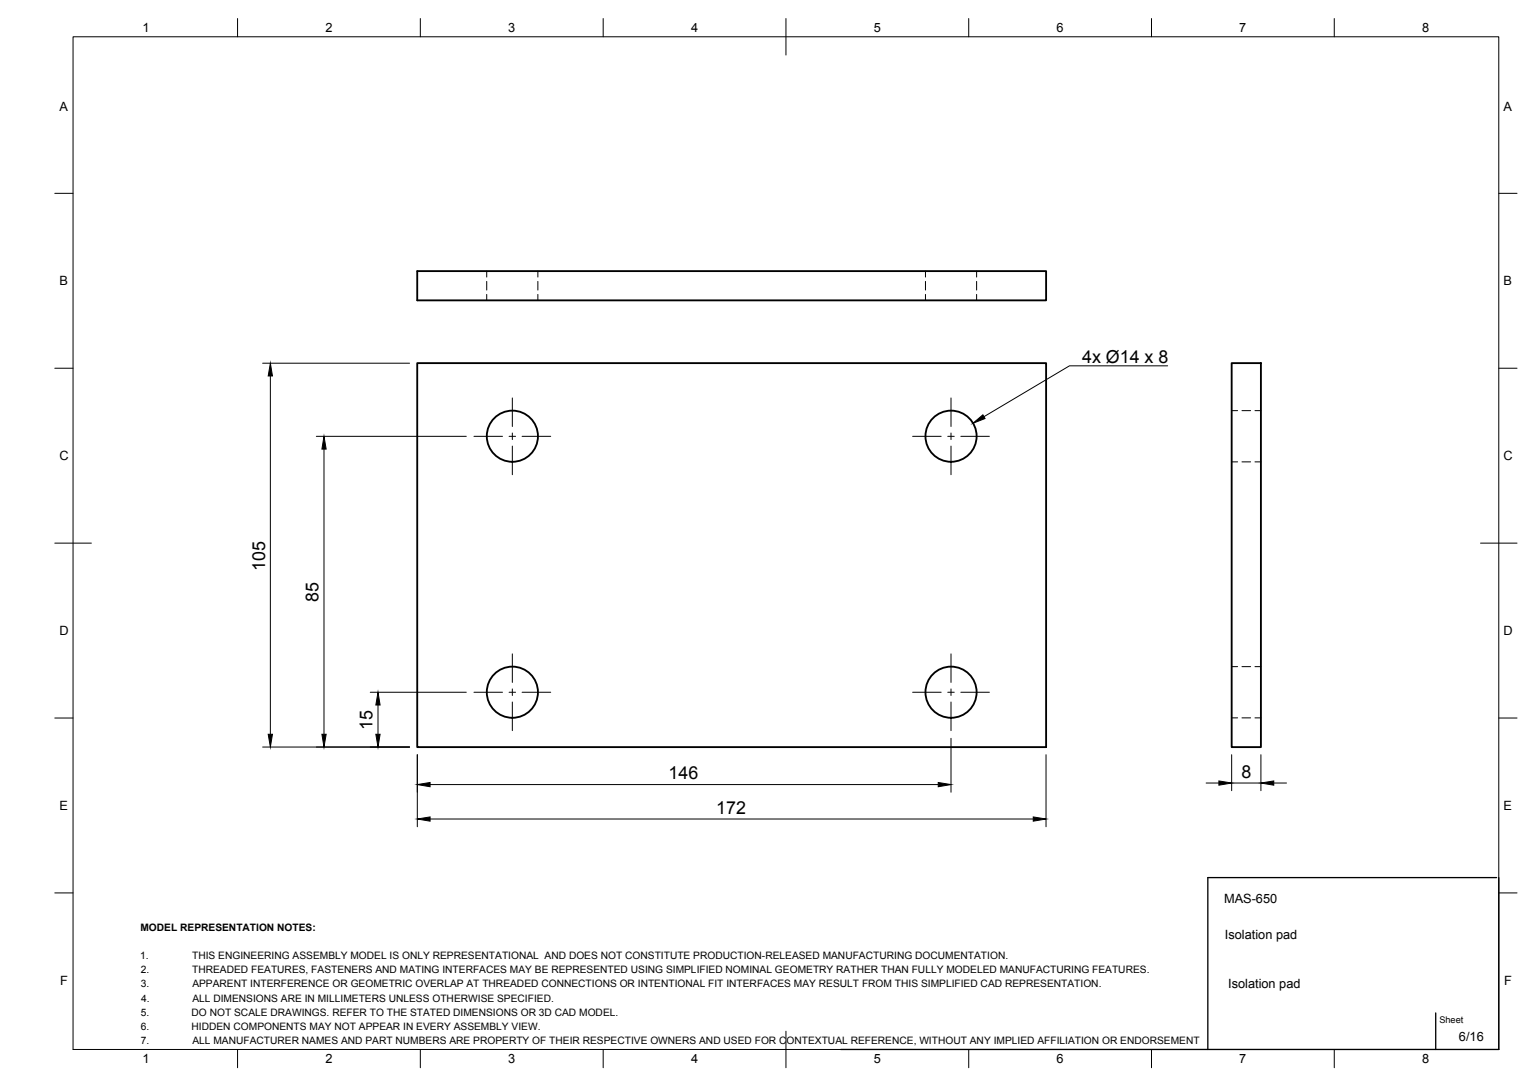
ISO-10303-21;
HEADER;
/* Generated by software containing ST-Developer
 * from STEP Tools, Inc. (www.steptools.com) 
 */

FILE_DESCRIPTION(
/* description */ ('Independent manual traversing gantry with native reusable aluminum pr
ofiles,180mm captured carriage travel, four bronze-bushed rollers, lin
ked ideal rolling motion, bonded acetal lateral guides, positive welde
d end stops and fully retained axle stacks. Editable native profile cu
t lengths220/400mm. Tool attachments viaM6 bridge-plate taps; mounted 
tool outside assembly. Welds, anchors, adhesives, fits, traction, load
/speed/structural/life ratings unassigned.'),
/* implementation_level */ '2;1');

FILE_NAME(
/* name */ 'Isolation pad.step',
/* time_stamp */ '2026-11-09T20:04:38-08:00',
/* author */ (''),
/* organization */ (''),
/* preprocessor_version */ 'ST-DEVELOPER v20.2',
/* originating_system */ 'Autodesk Translation Framework v15.17.0.0',
/* authorisation */ '');

FILE_SCHEMA (('AUTOMOTIVE_DESIGN { 1 0 10303 214 3 1 1 }'));
ENDSEC;

DATA;
#10=MECHANICAL_DESIGN_GEOMETRIC_PRESENTATION_REPRESENTATION('',(#474),#13231);
#442=SHAPE_REPRESENTATION_RELATIONSHIP('SRR','None',#13331,#458);
#458=ADVANCED_BREP_SHAPE_REPRESENTATION('',(#490),#13218);
#474=STYLED_ITEM('',(#13420),#490);
#490=MANIFOLD_SOLID_BREP('Body1',#4154);
#515=FACE_BOUND('',#921,.T.);
#516=FACE_BOUND('',#922,.T.);
#517=FACE_BOUND('',#923,.T.);
#518=FACE_BOUND('',#924,.T.);
#519=FACE_BOUND('',#926,.T.);
#520=FACE_BOUND('',#927,.T.);
#521=FACE_BOUND('',#928,.T.);
#522=FACE_BOUND('',#929,.T.);
#578=PLANE('',#4447);
#579=PLANE('',#4448);
#580=PLANE('',#4449);
#581=PLANE('',#4450);
#582=PLANE('',#4451);
#583=PLANE('',#4452);
#679=FACE_OUTER_BOUND('',#912,.T.);
#680=FACE_OUTER_BOUND('',#913,.T.);
#681=FACE_OUTER_BOUND('',#914,.T.);
#682=FACE_OUTER_BOUND('',#915,.T.);
#683=FACE_OUTER_BOUND('',#916,.T.);
#684=FACE_OUTER_BOUND('',#917,.T.);
#685=FACE_OUTER_BOUND('',#918,.T.);
#686=FACE_OUTER_BOUND('',#919,.T.);
#687=FACE_OUTER_BOUND('',#920,.T.);
#688=FACE_OUTER_BOUND('',#925,.T.);
#912=EDGE_LOOP('',(#2922,#2923,#2924,#2925));
#913=EDGE_LOOP('',(#2926,#2927,#2928,#2929));
#914=EDGE_LOOP('',(#2930,#2931,#2932,#2933));
#915=EDGE_LOOP('',(#2934,#2935,#2936,#2937));
#916=EDGE_LOOP('',(#2938,#2939,#2940,#2941));
#917=EDGE_LOOP('',(#2942,#2943,#2944,#2945));
#918=EDGE_LOOP('',(#2946,#2947,#2948,#2949));
#919=EDGE_LOOP('',(#2950,#2951,#2952,#2953));
#920=EDGE_LOOP('',(#2954,#2955,#2956,#2957));
#921=EDGE_LOOP('',(#2958));
#922=EDGE_LOOP('',(#2959));
#923=EDGE_LOOP('',(#2960));
#924=EDGE_LOOP('',(#2961));
#925=EDGE_LOOP('',(#2962,#2963,#2964,#2965));
#926=EDGE_LOOP('',(#2966));
#927=EDGE_LOOP('',(#2967));
#928=EDGE_LOOP('',(#2968));
#929=EDGE_LOOP('',(#2969));
#1204=LINE('',#6034,#1466);
#1205=LINE('',#6040,#1467);
#1206=LINE('',#6046,#1468);
#1207=LINE('',#6052,#1469);
#1208=LINE('',#6057,#1470);
#1209=LINE('',#6059,#1471);
#1210=LINE('',#6061,#1472);
#1211=LINE('',#6062,#1473);
#1212=LINE('',#6065,#1474);
#1213=LINE('',#6067,#1475);
#1214=LINE('',#6068,#1476);
#1215=LINE('',#6071,#1477);
#1216=LINE('',#6073,#1478);
#1217=LINE('',#6074,#1479);
#1218=LINE('',#6076,#1480);
#1219=LINE('',#6077,#1481);
#1466=VECTOR('',#5001,7.);
#1467=VECTOR('',#5008,7.);
#1468=VECTOR('',#5015,7.);
#1469=VECTOR('',#5022,7.);
#1470=VECTOR('',#5027,10.);
#1471=VECTOR('',#5028,10.);
#1472=VECTOR('',#5029,10.);
#1473=VECTOR('',#5030,10.);
#1474=VECTOR('',#5033,10.);
#1475=VECTOR('',#5034,10.);
#1476=VECTOR('',#5035,10.);
#1477=VECTOR('',#5038,10.);
#1478=VECTOR('',#5039,10.);
#1479=VECTOR('',#5040,10.);
#1480=VECTOR('',#5043,10.);
#1481=VECTOR('',#5044,10.);
#1688=CIRCLE('',#4436,7.);
#1689=CIRCLE('',#4437,7.);
#1690=CIRCLE('',#4439,7.);
#1691=CIRCLE('',#4440,7.);
#1692=CIRCLE('',#4442,7.);
#1693=CIRCLE('',#4443,7.);
#1694=CIRCLE('',#4445,7.);
#1695=CIRCLE('',#4446,7.);
#1832=VERTEX_POINT('',#6031);
#1833=VERTEX_POINT('',#6033);
#1834=VERTEX_POINT('',#6037);
#1835=VERTEX_POINT('',#6039);
#1836=VERTEX_POINT('',#6043);
#1837=VERTEX_POINT('',#6045);
#1838=VERTEX_POINT('',#6049);
#1839=VERTEX_POINT('',#6051);
#1840=VERTEX_POINT('',#6055);
#1841=VERTEX_POINT('',#6056);
#1842=VERTEX_POINT('',#6058);
#1843=VERTEX_POINT('',#6060);
#1844=VERTEX_POINT('',#6064);
#1845=VERTEX_POINT('',#6066);
#1846=VERTEX_POINT('',#6070);
#1847=VERTEX_POINT('',#6072);
#2244=EDGE_CURVE('',#1832,#1832,#1688,.T.);
#2245=EDGE_CURVE('',#1832,#1833,#1204,.T.);
#2246=EDGE_CURVE('',#1833,#1833,#1689,.T.);
#2247=EDGE_CURVE('',#1834,#1834,#1690,.T.);
#2248=EDGE_CURVE('',#1834,#1835,#1205,.T.);
#2249=EDGE_CURVE('',#1835,#1835,#1691,.T.);
#2250=EDGE_CURVE('',#1836,#1836,#1692,.T.);
#2251=EDGE_CURVE('',#1836,#1837,#1206,.T.);
#2252=EDGE_CURVE('',#1837,#1837,#1693,.T.);
#2253=EDGE_CURVE('',#1838,#1838,#1694,.T.);
#2254=EDGE_CURVE('',#1838,#1839,#1207,.T.);
#2255=EDGE_CURVE('',#1839,#1839,#1695,.T.);
#2256=EDGE_CURVE('',#1840,#1841,#1208,.F.);
#2257=EDGE_CURVE('',#1841,#1842,#1209,.T.);
#2258=EDGE_CURVE('',#1843,#1842,#1210,.F.);
#2259=EDGE_CURVE('',#1840,#1843,#1211,.T.);
#2260=EDGE_CURVE('',#1844,#1840,#1212,.F.);
#2261=EDGE_CURVE('',#1845,#1843,#1213,.F.);
#2262=EDGE_CURVE('',#1844,#1845,#1214,.T.);
#2263=EDGE_CURVE('',#1846,#1844,#1215,.F.);
#2264=EDGE_CURVE('',#1847,#1845,#1216,.F.);
#2265=EDGE_CURVE('',#1846,#1847,#1217,.F.);
#2266=EDGE_CURVE('',#1841,#1846,#1218,.T.);
#2267=EDGE_CURVE('',#1842,#1847,#1219,.T.);
#2922=ORIENTED_EDGE('',*,*,#2244,.F.);
#2923=ORIENTED_EDGE('',*,*,#2245,.T.);
#2924=ORIENTED_EDGE('',*,*,#2246,.F.);
#2925=ORIENTED_EDGE('',*,*,#2245,.F.);
#2926=ORIENTED_EDGE('',*,*,#2247,.F.);
#2927=ORIENTED_EDGE('',*,*,#2248,.T.);
#2928=ORIENTED_EDGE('',*,*,#2249,.F.);
#2929=ORIENTED_EDGE('',*,*,#2248,.F.);
#2930=ORIENTED_EDGE('',*,*,#2250,.F.);
#2931=ORIENTED_EDGE('',*,*,#2251,.T.);
#2932=ORIENTED_EDGE('',*,*,#2252,.F.);
#2933=ORIENTED_EDGE('',*,*,#2251,.F.);
#2934=ORIENTED_EDGE('',*,*,#2253,.F.);
#2935=ORIENTED_EDGE('',*,*,#2254,.T.);
#2936=ORIENTED_EDGE('',*,*,#2255,.F.);
#2937=ORIENTED_EDGE('',*,*,#2254,.F.);
#2938=ORIENTED_EDGE('',*,*,#2256,.T.);
#2939=ORIENTED_EDGE('',*,*,#2257,.T.);
#2940=ORIENTED_EDGE('',*,*,#2258,.F.);
#2941=ORIENTED_EDGE('',*,*,#2259,.F.);
#2942=ORIENTED_EDGE('',*,*,#2260,.T.);
#2943=ORIENTED_EDGE('',*,*,#2259,.T.);
#2944=ORIENTED_EDGE('',*,*,#2261,.F.);
#2945=ORIENTED_EDGE('',*,*,#2262,.F.);
#2946=ORIENTED_EDGE('',*,*,#2263,.T.);
#2947=ORIENTED_EDGE('',*,*,#2262,.T.);
#2948=ORIENTED_EDGE('',*,*,#2264,.F.);
#2949=ORIENTED_EDGE('',*,*,#2265,.F.);
#2950=ORIENTED_EDGE('',*,*,#2266,.T.);
#2951=ORIENTED_EDGE('',*,*,#2265,.T.);
#2952=ORIENTED_EDGE('',*,*,#2267,.F.);
#2953=ORIENTED_EDGE('',*,*,#2257,.F.);
#2954=ORIENTED_EDGE('',*,*,#2267,.T.);
#2955=ORIENTED_EDGE('',*,*,#2264,.T.);
#2956=ORIENTED_EDGE('',*,*,#2261,.T.);
#2957=ORIENTED_EDGE('',*,*,#2258,.T.);
#2958=ORIENTED_EDGE('',*,*,#2244,.T.);
#2959=ORIENTED_EDGE('',*,*,#2247,.T.);
#2960=ORIENTED_EDGE('',*,*,#2250,.T.);
#2961=ORIENTED_EDGE('',*,*,#2253,.T.);
#2962=ORIENTED_EDGE('',*,*,#2266,.F.);
#2963=ORIENTED_EDGE('',*,*,#2256,.F.);
#2964=ORIENTED_EDGE('',*,*,#2260,.F.);
#2965=ORIENTED_EDGE('',*,*,#2263,.F.);
#2966=ORIENTED_EDGE('',*,*,#2246,.T.);
#2967=ORIENTED_EDGE('',*,*,#2249,.T.);
#2968=ORIENTED_EDGE('',*,*,#2252,.T.);
#2969=ORIENTED_EDGE('',*,*,#2255,.T.);
#3818=CYLINDRICAL_SURFACE('',#4435,7.);
#3819=CYLINDRICAL_SURFACE('',#4438,7.);
#3820=CYLINDRICAL_SURFACE('',#4441,7.);
#3821=CYLINDRICAL_SURFACE('',#4444,7.);
#3976=ADVANCED_FACE('',(#679),#3818,.F.);
#3977=ADVANCED_FACE('',(#680),#3819,.F.);
#3978=ADVANCED_FACE('',(#681),#3820,.F.);
#3979=ADVANCED_FACE('',(#682),#3821,.F.);
#3980=ADVANCED_FACE('',(#683),#578,.T.);
#3981=ADVANCED_FACE('',(#684),#579,.T.);
#3982=ADVANCED_FACE('',(#685),#580,.T.);
#3983=ADVANCED_FACE('',(#686),#581,.T.);
#3984=ADVANCED_FACE('',(#687,#515,#516,#517,#518),#582,.T.);
#3985=ADVANCED_FACE('',(#688,#519,#520,#521,#522),#583,.F.);
#4154=CLOSED_SHELL('',(#3976,#3977,#3978,#3979,#3980,#3981,#3982,#3983,
#3984,#3985));
#4434=AXIS2_PLACEMENT_3D('',#6029,#4995,#4996);
#4435=AXIS2_PLACEMENT_3D('',#6030,#4997,#4998);
#4436=AXIS2_PLACEMENT_3D('',#6032,#4999,#5000);
#4437=AXIS2_PLACEMENT_3D('',#6035,#5002,#5003);
#4438=AXIS2_PLACEMENT_3D('',#6036,#5004,#5005);
#4439=AXIS2_PLACEMENT_3D('',#6038,#5006,#5007);
#4440=AXIS2_PLACEMENT_3D('',#6041,#5009,#5010);
#4441=AXIS2_PLACEMENT_3D('',#6042,#5011,#5012);
#4442=AXIS2_PLACEMENT_3D('',#6044,#5013,#5014);
#4443=AXIS2_PLACEMENT_3D('',#6047,#5016,#5017);
#4444=AXIS2_PLACEMENT_3D('',#6048,#5018,#5019);
#4445=AXIS2_PLACEMENT_3D('',#6050,#5020,#5021);
#4446=AXIS2_PLACEMENT_3D('',#6053,#5023,#5024);
#4447=AXIS2_PLACEMENT_3D('',#6054,#5025,#5026);
#4448=AXIS2_PLACEMENT_3D('',#6063,#5031,#5032);
#4449=AXIS2_PLACEMENT_3D('',#6069,#5036,#5037);
#4450=AXIS2_PLACEMENT_3D('',#6075,#5041,#5042);
#4451=AXIS2_PLACEMENT_3D('',#6078,#5045,#5046);
#4452=AXIS2_PLACEMENT_3D('',#6079,#5047,#5048);
#4995=DIRECTION('axis',(0.,0.,1.));
#4996=DIRECTION('refdir',(1.,0.,0.));
#4997=DIRECTION('center_axis',(0.,0.,-1.));
#4998=DIRECTION('ref_axis',(1.,0.,0.));
#4999=DIRECTION('center_axis',(0.,0.,-1.));
#5000=DIRECTION('ref_axis',(1.,0.,0.));
#5001=DIRECTION('',(0.,0.,-1.));
#5002=DIRECTION('center_axis',(0.,0.,1.));
#5003=DIRECTION('ref_axis',(1.,0.,0.));
#5004=DIRECTION('center_axis',(0.,0.,-1.));
#5005=DIRECTION('ref_axis',(1.,0.,0.));
#5006=DIRECTION('center_axis',(0.,0.,-1.));
#5007=DIRECTION('ref_axis',(1.,0.,0.));
#5008=DIRECTION('',(0.,0.,-1.));
#5009=DIRECTION('center_axis',(0.,0.,1.));
#5010=DIRECTION('ref_axis',(1.,0.,0.));
#5011=DIRECTION('center_axis',(0.,0.,-1.));
#5012=DIRECTION('ref_axis',(1.,0.,0.));
#5013=DIRECTION('center_axis',(0.,0.,-1.));
#5014=DIRECTION('ref_axis',(1.,0.,0.));
#5015=DIRECTION('',(0.,0.,-1.));
#5016=DIRECTION('center_axis',(0.,0.,1.));
#5017=DIRECTION('ref_axis',(1.,0.,0.));
#5018=DIRECTION('center_axis',(0.,0.,-1.));
#5019=DIRECTION('ref_axis',(1.,0.,0.));
#5020=DIRECTION('center_axis',(0.,0.,-1.));
#5021=DIRECTION('ref_axis',(1.,0.,0.));
#5022=DIRECTION('',(0.,0.,-1.));
#5023=DIRECTION('center_axis',(0.,0.,1.));
#5024=DIRECTION('ref_axis',(1.,0.,0.));
#5025=DIRECTION('center_axis',(0.,1.,0.));
#5026=DIRECTION('ref_axis',(-1.,0.,0.));
#5027=DIRECTION('',(1.,0.,0.));
#5028=DIRECTION('',(0.,0.,1.));
#5029=DIRECTION('',(1.,0.,0.));
#5030=DIRECTION('',(0.,0.,1.));
#5031=DIRECTION('center_axis',(1.,0.,0.));
#5032=DIRECTION('ref_axis',(0.,1.,0.));
#5033=DIRECTION('',(0.,-1.,0.));
#5034=DIRECTION('',(0.,-1.,0.));
#5035=DIRECTION('',(0.,0.,1.));
#5036=DIRECTION('center_axis',(0.,-1.,0.));
#5037=DIRECTION('ref_axis',(1.,0.,0.));
#5038=DIRECTION('',(-1.,0.,0.));
#5039=DIRECTION('',(-1.,0.,0.));
#5040=DIRECTION('',(0.,0.,-1.));
#5041=DIRECTION('center_axis',(-1.,0.,0.));
#5042=DIRECTION('ref_axis',(0.,-1.,0.));
#5043=DIRECTION('',(0.,-1.,0.));
#5044=DIRECTION('',(0.,-1.,0.));
#5045=DIRECTION('center_axis',(0.,0.,1.));
#5046=DIRECTION('ref_axis',(1.,0.,0.));
#5047=DIRECTION('center_axis',(0.,0.,1.));
#5048=DIRECTION('ref_axis',(1.,0.,0.));
#6029=CARTESIAN_POINT('',(0.,0.,0.));
#6030=CARTESIAN_POINT('Origin',(35.,-60.,4.));
#6031=CARTESIAN_POINT('',(28.,-60.,8.));
#6032=CARTESIAN_POINT('Origin',(35.,-60.,8.));
#6033=CARTESIAN_POINT('',(28.,-60.,0.));
#6034=CARTESIAN_POINT('',(28.,-60.,4.));
#6035=CARTESIAN_POINT('Origin',(35.,-60.,0.));
#6036=CARTESIAN_POINT('Origin',(-35.,-60.,4.));
#6037=CARTESIAN_POINT('',(-42.,-60.,8.));
#6038=CARTESIAN_POINT('Origin',(-35.,-60.,8.));
#6039=CARTESIAN_POINT('',(-42.,-60.,0.));
#6040=CARTESIAN_POINT('',(-42.,-60.,4.));
#6041=CARTESIAN_POINT('Origin',(-35.,-60.,0.));
#6042=CARTESIAN_POINT('Origin',(-35.,60.,4.));
#6043=CARTESIAN_POINT('',(-42.,60.,8.));
#6044=CARTESIAN_POINT('Origin',(-35.,60.,8.));
#6045=CARTESIAN_POINT('',(-42.,60.,0.));
#6046=CARTESIAN_POINT('',(-42.,60.,4.));
#6047=CARTESIAN_POINT('Origin',(-35.,60.,0.));
#6048=CARTESIAN_POINT('Origin',(35.,60.,4.));
#6049=CARTESIAN_POINT('',(28.,60.,8.));
#6050=CARTESIAN_POINT('Origin',(35.,60.,8.));
#6051=CARTESIAN_POINT('',(28.,60.,0.));
#6052=CARTESIAN_POINT('',(28.,60.,4.));
#6053=CARTESIAN_POINT('Origin',(35.,60.,0.));
#6054=CARTESIAN_POINT('Origin',(50.,86.,0.));
#6055=CARTESIAN_POINT('',(55.,86.,0.));
#6056=CARTESIAN_POINT('',(-50.,86.,0.));
#6057=CARTESIAN_POINT('',(25.,86.,0.));
#6058=CARTESIAN_POINT('',(-50.,86.,8.));
#6059=CARTESIAN_POINT('',(-50.,86.,0.));
#6060=CARTESIAN_POINT('',(55.,86.,8.));
#6061=CARTESIAN_POINT('',(25.,86.,8.));
#6062=CARTESIAN_POINT('',(55.,86.,0.));
#6063=CARTESIAN_POINT('Origin',(55.,-80.,0.));
#6064=CARTESIAN_POINT('',(55.,-86.,0.));
#6065=CARTESIAN_POINT('',(55.,-40.,0.));
#6066=CARTESIAN_POINT('',(55.,-86.,8.));
#6067=CARTESIAN_POINT('',(55.,-40.,8.));
#6068=CARTESIAN_POINT('',(55.,-86.,0.));
#6069=CARTESIAN_POINT('Origin',(-50.,-86.,0.));
#6070=CARTESIAN_POINT('',(-50.,-86.,0.));
#6071=CARTESIAN_POINT('',(-25.,-86.,0.));
#6072=CARTESIAN_POINT('',(-50.,-86.,8.));
#6073=CARTESIAN_POINT('',(-25.,-86.,8.));
#6074=CARTESIAN_POINT('',(-50.,-86.,0.));
#6075=CARTESIAN_POINT('Origin',(-50.,80.,0.));
#6076=CARTESIAN_POINT('',(-50.,80.,0.));
#6077=CARTESIAN_POINT('',(-50.,80.,8.));
#6078=CARTESIAN_POINT('Origin',(0.,0.,8.));
#6079=CARTESIAN_POINT('Origin',(0.,0.,0.));
#13200=UNCERTAINTY_MEASURE_WITH_UNIT(LENGTH_MEASURE(0.01),#13232,
'DISTANCE_ACCURACY_VALUE',
'Maximum model space distance between geometric entities at asserted c
onnectivities');
#13213=UNCERTAINTY_MEASURE_WITH_UNIT(LENGTH_MEASURE(0.01),#13232,
'DISTANCE_ACCURACY_VALUE',
'Maximum model space distance between geometric entities at asserted c
onnectivities');
#13218=(
GEOMETRIC_REPRESENTATION_CONTEXT(3)
GLOBAL_UNCERTAINTY_ASSIGNED_CONTEXT((#13200))
GLOBAL_UNIT_ASSIGNED_CONTEXT((#13232,#13234,#13235))
REPRESENTATION_CONTEXT('','3D')
);
#13231=(
GEOMETRIC_REPRESENTATION_CONTEXT(3)
GLOBAL_UNCERTAINTY_ASSIGNED_CONTEXT((#13213))
GLOBAL_UNIT_ASSIGNED_CONTEXT((#13232,#13234,#13235))
REPRESENTATION_CONTEXT('','3D')
);
#13232=(
LENGTH_UNIT()
NAMED_UNIT(*)
SI_UNIT(.MILLI.,.METRE.)
);
#13234=(
NAMED_UNIT(*)
PLANE_ANGLE_UNIT()
SI_UNIT($,.RADIAN.)
);
#13235=(
NAMED_UNIT(*)
SI_UNIT($,.STERADIAN.)
SOLID_ANGLE_UNIT()
);
#13240=SHAPE_DEFINITION_REPRESENTATION(#13257,#13331);
#13257=PRODUCT_DEFINITION_SHAPE('',$,#13349);
#13331=SHAPE_REPRESENTATION('',(#4434),#13218);
#13344=PRODUCT_DEFINITION_CONTEXT('part definition',#13397,'design');
#13349=PRODUCT_DEFINITION('Isolation pad','Isolation pad',#13366,#13344);
#13366=PRODUCT_DEFINITION_FORMATION('',$,#13403);
#13397=APPLICATION_CONTEXT(
'Core Data for Automotive Mechanical Design Process');
#13398=PRODUCT_CONTEXT('part definition',#13397,'mechanical');
#13403=PRODUCT('Isolation pad','Isolation pad',$,(#13398));
#13420=PRESENTATION_STYLE_ASSIGNMENT((#13434));
#13434=SURFACE_STYLE_USAGE(.BOTH.,#13448);
#13448=SURFACE_SIDE_STYLE('',(#13462));
#13462=SURFACE_STYLE_FILL_AREA(#13476);
#13476=FILL_AREA_STYLE('Charcoal',(#13490));
#13490=FILL_AREA_STYLE_COLOUR('Charcoal',#13504);
#13504=COLOUR_RGB('Charcoal',0.164705882352941,0.184313725490196,0.211764705882353);
ENDSEC;
END-ISO-10303-21;
